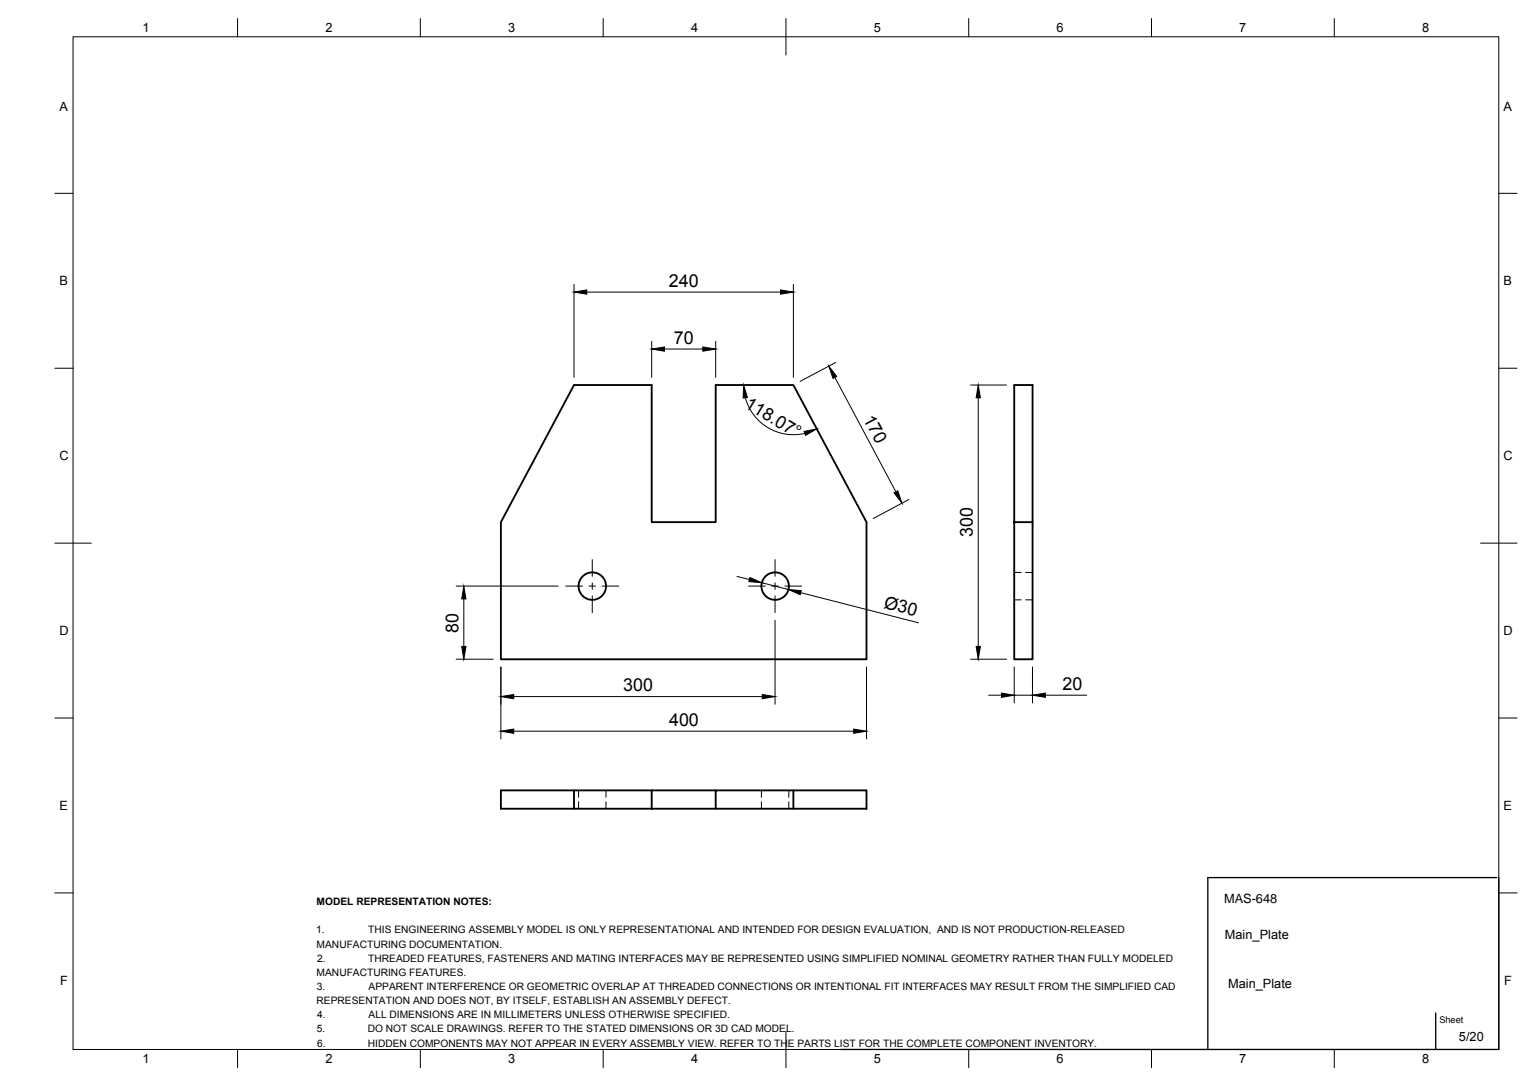
ISO-10303-21;
HEADER;
FILE_DESCRIPTION((''),'2;1');
FILE_NAME('Main_Plate.step','2026-10-09T12:47:58-07:00',(''),(''),'','','');
FILE_SCHEMA (('AUTOMOTIVE_DESIGN { 1 0 10303 214 3 1 1 }'));
ENDSEC;
DATA;
#10=MECHANICAL_DESIGN_GEOMETRIC_PRESENTATION_REPRESENTATION('',(#312),#3475);
#143=FACE_BOUND('',#473,.T.) ;
#144=FACE_BOUND('',#474,.T.) ;
#145=FACE_BOUND('',#476,.T.) ;
#146=FACE_BOUND('',#477,.T.) ;
#168=CIRCLE('',#1990,15.) ;
#169=CIRCLE('',#1991,15.) ;
#170=CIRCLE('',#1993,15.) ;
#171=CIRCLE('',#1994,15.) ;
#257=CYLINDRICAL_SURFACE('',#1989,15.) ;
#258=CYLINDRICAL_SURFACE('',#1992,15.) ;
#288=SHAPE_REPRESENTATION_RELATIONSHIP('SRR','None',#3542,#300) ;
#300=ADVANCED_BREP_SHAPE_REPRESENTATION('',(#324),#3462) ;
#312=STYLED_ITEM('',(#3628),#324) ;
#324=MANIFOLD_SOLID_BREP('Body1',#1826) ;
#347=FACE_OUTER_BOUND('',#463,.T.) ;
#348=FACE_OUTER_BOUND('',#464,.T.) ;
#349=FACE_OUTER_BOUND('',#465,.T.) ;
#350=FACE_OUTER_BOUND('',#466,.T.) ;
#351=FACE_OUTER_BOUND('',#467,.T.) ;
#352=FACE_OUTER_BOUND('',#468,.T.) ;
#353=FACE_OUTER_BOUND('',#469,.T.) ;
#354=FACE_OUTER_BOUND('',#470,.T.) ;
#355=FACE_OUTER_BOUND('',#471,.T.) ;
#356=FACE_OUTER_BOUND('',#472,.T.) ;
#357=FACE_OUTER_BOUND('',#475,.T.) ;
#358=FACE_OUTER_BOUND('',#478,.T.) ;
#359=FACE_OUTER_BOUND('',#479,.T.) ;
#360=FACE_OUTER_BOUND('',#480,.T.) ;
#463=EDGE_LOOP('',(#1248,#1249,#1250,#1251)) ;
#464=EDGE_LOOP('',(#1252,#1253,#1254,#1255)) ;
#465=EDGE_LOOP('',(#1256,#1257,#1258,#1259)) ;
#466=EDGE_LOOP('',(#1260,#1261,#1262,#1263)) ;
#467=EDGE_LOOP('',(#1264,#1265,#1266,#1267)) ;
#468=EDGE_LOOP('',(#1268,#1269,#1270,#1271)) ;
#469=EDGE_LOOP('',(#1272,#1273,#1274,#1275)) ;
#470=EDGE_LOOP('',(#1276,#1277,#1278,#1279)) ;
#471=EDGE_LOOP('',(#1280,#1281,#1282,#1283)) ;
#472=EDGE_LOOP('',(#1284,#1285,#1286,#1287,#1288,#1289,#1290,#1291,#1292,
#1293)) ;
#473=EDGE_LOOP('',(#1294)) ;
#474=EDGE_LOOP('',(#1295)) ;
#475=EDGE_LOOP('',(#1296,#1297,#1298,#1299,#1300,#1301,#1302,#1303,#1304,
#1305)) ;
#476=EDGE_LOOP('',(#1306)) ;
#477=EDGE_LOOP('',(#1307)) ;
#478=EDGE_LOOP('',(#1308,#1309,#1310,#1311)) ;
#479=EDGE_LOOP('',(#1312,#1313,#1314,#1315)) ;
#480=EDGE_LOOP('',(#1316,#1317,#1318,#1319)) ;
#612=LINE('',#2890,#731) ;
#613=LINE('',#2896,#732) ;
#614=LINE('',#2901,#733) ;
#615=LINE('',#2903,#734) ;
#616=LINE('',#2905,#735) ;
#617=LINE('',#2906,#736) ;
#618=LINE('',#2910,#737) ;
#619=LINE('',#2912,#738) ;
#620=LINE('',#2914,#739) ;
#621=LINE('',#2915,#740) ;
#622=LINE('',#2918,#741) ;
#623=LINE('',#2920,#742) ;
#624=LINE('',#2921,#743) ;
#625=LINE('',#2924,#744) ;
#626=LINE('',#2926,#745) ;
#627=LINE('',#2927,#746) ;
#628=LINE('',#2930,#747) ;
#629=LINE('',#2932,#748) ;
#630=LINE('',#2933,#749) ;
#631=LINE('',#2937,#750) ;
#632=LINE('',#2938,#751) ;
#633=LINE('',#2939,#752) ;
#634=LINE('',#2941,#753) ;
#635=LINE('',#2942,#754) ;
#636=LINE('',#2946,#755) ;
#637=LINE('',#2947,#756) ;
#638=LINE('',#2948,#757) ;
#639=LINE('',#2951,#758) ;
#640=LINE('',#2953,#759) ;
#641=LINE('',#2954,#760) ;
#642=LINE('',#2956,#761) ;
#643=LINE('',#2957,#762) ;
#731=VECTOR('',#2283,15.) ;
#732=VECTOR('',#2290,15.) ;
#733=VECTOR('',#2295,1000.) ;
#734=VECTOR('',#2296,1000.) ;
#735=VECTOR('',#2297,1000.) ;
#736=VECTOR('',#2298,1000.) ;
#737=VECTOR('',#2301,1000.) ;
#738=VECTOR('',#2302,1000.) ;
#739=VECTOR('',#2303,1000.) ;
#740=VECTOR('',#2304,1000.) ;
#741=VECTOR('',#2307,1000.) ;
#742=VECTOR('',#2308,1000.) ;
#743=VECTOR('',#2309,1000.) ;
#744=VECTOR('',#2312,1000.) ;
#745=VECTOR('',#2313,1000.) ;
#746=VECTOR('',#2314,1000.) ;
#747=VECTOR('',#2317,1000.) ;
#748=VECTOR('',#2318,1000.) ;
#749=VECTOR('',#2319,1000.) ;
#750=VECTOR('',#2322,1000.) ;
#751=VECTOR('',#2323,1000.) ;
#752=VECTOR('',#2324,1000.) ;
#753=VECTOR('',#2327,1000.) ;
#754=VECTOR('',#2328,1000.) ;
#755=VECTOR('',#2331,1000.) ;
#756=VECTOR('',#2332,1000.) ;
#757=VECTOR('',#2333,1000.) ;
#758=VECTOR('',#2336,1000.) ;
#759=VECTOR('',#2337,1000.) ;
#760=VECTOR('',#2338,1000.) ;
#761=VECTOR('',#2341,1000.) ;
#762=VECTOR('',#2342,1000.) ;
#843=VERTEX_POINT('',#2887) ;
#844=VERTEX_POINT('',#2889) ;
#845=VERTEX_POINT('',#2893) ;
#846=VERTEX_POINT('',#2895) ;
#847=VERTEX_POINT('',#2899) ;
#848=VERTEX_POINT('',#2900) ;
#849=VERTEX_POINT('',#2902) ;
#850=VERTEX_POINT('',#2904) ;
#851=VERTEX_POINT('',#2908) ;
#852=VERTEX_POINT('',#2909) ;
#853=VERTEX_POINT('',#2911) ;
#854=VERTEX_POINT('',#2913) ;
#855=VERTEX_POINT('',#2917) ;
#856=VERTEX_POINT('',#2919) ;
#857=VERTEX_POINT('',#2923) ;
#858=VERTEX_POINT('',#2925) ;
#859=VERTEX_POINT('',#2929) ;
#860=VERTEX_POINT('',#2931) ;
#861=VERTEX_POINT('',#2935) ;
#862=VERTEX_POINT('',#2936) ;
#863=VERTEX_POINT('',#2944) ;
#864=VERTEX_POINT('',#2945) ;
#865=VERTEX_POINT('',#2950) ;
#866=VERTEX_POINT('',#2952) ;
#996=EDGE_CURVE('',#843,#843,#168,.T.) ;
#997=EDGE_CURVE('',#843,#844,#612,.T.) ;
#998=EDGE_CURVE('',#844,#844,#169,.T.) ;
#999=EDGE_CURVE('',#845,#845,#170,.T.) ;
#1000=EDGE_CURVE('',#845,#846,#613,.T.) ;
#1001=EDGE_CURVE('',#846,#846,#171,.T.) ;
#1002=EDGE_CURVE('',#847,#848,#614,.T.) ;
#1003=EDGE_CURVE('',#849,#847,#615,.T.) ;
#1004=EDGE_CURVE('',#850,#849,#616,.T.) ;
#1005=EDGE_CURVE('',#850,#848,#617,.T.) ;
#1006=EDGE_CURVE('',#851,#852,#618,.T.) ;
#1007=EDGE_CURVE('',#853,#851,#619,.T.) ;
#1008=EDGE_CURVE('',#853,#854,#620,.T.) ;
#1009=EDGE_CURVE('',#854,#852,#621,.T.) ;
#1010=EDGE_CURVE('',#855,#851,#622,.T.) ;
#1011=EDGE_CURVE('',#856,#855,#623,.T.) ;
#1012=EDGE_CURVE('',#856,#853,#624,.T.) ;
#1013=EDGE_CURVE('',#857,#855,#625,.T.) ;
#1014=EDGE_CURVE('',#858,#857,#626,.T.) ;
#1015=EDGE_CURVE('',#858,#856,#627,.T.) ;
#1016=EDGE_CURVE('',#859,#857,#628,.T.) ;
#1017=EDGE_CURVE('',#860,#859,#629,.T.) ;
#1018=EDGE_CURVE('',#860,#858,#630,.T.) ;
#1019=EDGE_CURVE('',#861,#862,#631,.T.) ;
#1020=EDGE_CURVE('',#861,#860,#632,.T.) ;
#1021=EDGE_CURVE('',#862,#859,#633,.T.) ;
#1022=EDGE_CURVE('',#852,#849,#634,.T.) ;
#1023=EDGE_CURVE('',#854,#850,#635,.T.) ;
#1024=EDGE_CURVE('',#863,#864,#636,.T.) ;
#1025=EDGE_CURVE('',#864,#848,#637,.T.) ;
#1026=EDGE_CURVE('',#861,#863,#638,.T.) ;
#1027=EDGE_CURVE('',#865,#847,#639,.T.) ;
#1028=EDGE_CURVE('',#866,#865,#640,.T.) ;
#1029=EDGE_CURVE('',#862,#866,#641,.T.) ;
#1030=EDGE_CURVE('',#863,#866,#642,.T.) ;
#1031=EDGE_CURVE('',#864,#865,#643,.T.) ;
#1248=ORIENTED_EDGE('',*,*,#996,.F.) ;
#1249=ORIENTED_EDGE('',*,*,#997,.T.) ;
#1250=ORIENTED_EDGE('',*,*,#998,.T.) ;
#1251=ORIENTED_EDGE('',*,*,#997,.F.) ;
#1252=ORIENTED_EDGE('',*,*,#999,.F.) ;
#1253=ORIENTED_EDGE('',*,*,#1000,.T.) ;
#1254=ORIENTED_EDGE('',*,*,#1001,.T.) ;
#1255=ORIENTED_EDGE('',*,*,#1000,.F.) ;
#1256=ORIENTED_EDGE('',*,*,#1002,.F.) ;
#1257=ORIENTED_EDGE('',*,*,#1003,.F.) ;
#1258=ORIENTED_EDGE('',*,*,#1004,.F.) ;
#1259=ORIENTED_EDGE('',*,*,#1005,.T.) ;
#1260=ORIENTED_EDGE('',*,*,#1006,.F.) ;
#1261=ORIENTED_EDGE('',*,*,#1007,.F.) ;
#1262=ORIENTED_EDGE('',*,*,#1008,.T.) ;
#1263=ORIENTED_EDGE('',*,*,#1009,.T.) ;
#1264=ORIENTED_EDGE('',*,*,#1010,.F.) ;
#1265=ORIENTED_EDGE('',*,*,#1011,.F.) ;
#1266=ORIENTED_EDGE('',*,*,#1012,.T.) ;
#1267=ORIENTED_EDGE('',*,*,#1007,.T.) ;
#1268=ORIENTED_EDGE('',*,*,#1013,.F.) ;
#1269=ORIENTED_EDGE('',*,*,#1014,.F.) ;
#1270=ORIENTED_EDGE('',*,*,#1015,.T.) ;
#1271=ORIENTED_EDGE('',*,*,#1011,.T.) ;
#1272=ORIENTED_EDGE('',*,*,#1016,.F.) ;
#1273=ORIENTED_EDGE('',*,*,#1017,.F.) ;
#1274=ORIENTED_EDGE('',*,*,#1018,.T.) ;
#1275=ORIENTED_EDGE('',*,*,#1014,.T.) ;
#1276=ORIENTED_EDGE('',*,*,#1019,.F.) ;
#1277=ORIENTED_EDGE('',*,*,#1020,.T.) ;
#1278=ORIENTED_EDGE('',*,*,#1017,.T.) ;
#1279=ORIENTED_EDGE('',*,*,#1021,.F.) ;
#1280=ORIENTED_EDGE('',*,*,#1022,.F.) ;
#1281=ORIENTED_EDGE('',*,*,#1009,.F.) ;
#1282=ORIENTED_EDGE('',*,*,#1023,.T.) ;
#1283=ORIENTED_EDGE('',*,*,#1004,.T.) ;
#1284=ORIENTED_EDGE('',*,*,#1024,.T.) ;
#1285=ORIENTED_EDGE('',*,*,#1025,.T.) ;
#1286=ORIENTED_EDGE('',*,*,#1005,.F.) ;
#1287=ORIENTED_EDGE('',*,*,#1023,.F.) ;
#1288=ORIENTED_EDGE('',*,*,#1008,.F.) ;
#1289=ORIENTED_EDGE('',*,*,#1012,.F.) ;
#1290=ORIENTED_EDGE('',*,*,#1015,.F.) ;
#1291=ORIENTED_EDGE('',*,*,#1018,.F.) ;
#1292=ORIENTED_EDGE('',*,*,#1020,.F.) ;
#1293=ORIENTED_EDGE('',*,*,#1026,.T.) ;
#1294=ORIENTED_EDGE('',*,*,#996,.T.) ;
#1295=ORIENTED_EDGE('',*,*,#999,.T.) ;
#1296=ORIENTED_EDGE('',*,*,#1027,.F.) ;
#1297=ORIENTED_EDGE('',*,*,#1028,.F.) ;
#1298=ORIENTED_EDGE('',*,*,#1029,.F.) ;
#1299=ORIENTED_EDGE('',*,*,#1021,.T.) ;
#1300=ORIENTED_EDGE('',*,*,#1016,.T.) ;
#1301=ORIENTED_EDGE('',*,*,#1013,.T.) ;
#1302=ORIENTED_EDGE('',*,*,#1010,.T.) ;
#1303=ORIENTED_EDGE('',*,*,#1006,.T.) ;
#1304=ORIENTED_EDGE('',*,*,#1022,.T.) ;
#1305=ORIENTED_EDGE('',*,*,#1003,.T.) ;
#1306=ORIENTED_EDGE('',*,*,#998,.F.) ;
#1307=ORIENTED_EDGE('',*,*,#1001,.F.) ;
#1308=ORIENTED_EDGE('',*,*,#1030,.T.) ;
#1309=ORIENTED_EDGE('',*,*,#1028,.T.) ;
#1310=ORIENTED_EDGE('',*,*,#1031,.F.) ;
#1311=ORIENTED_EDGE('',*,*,#1024,.F.) ;
#1312=ORIENTED_EDGE('',*,*,#1002,.T.) ;
#1313=ORIENTED_EDGE('',*,*,#1025,.F.) ;
#1314=ORIENTED_EDGE('',*,*,#1031,.T.) ;
#1315=ORIENTED_EDGE('',*,*,#1027,.T.) ;
#1316=ORIENTED_EDGE('',*,*,#1019,.T.) ;
#1317=ORIENTED_EDGE('',*,*,#1029,.T.) ;
#1318=ORIENTED_EDGE('',*,*,#1030,.F.) ;
#1319=ORIENTED_EDGE('',*,*,#1026,.F.) ;
#1656=PLANE('',#1995) ;
#1657=PLANE('',#1996) ;
#1658=PLANE('',#1997) ;
#1659=PLANE('',#1998) ;
#1660=PLANE('',#1999) ;
#1661=PLANE('',#2000) ;
#1662=PLANE('',#2001) ;
#1663=PLANE('',#2002) ;
#1664=PLANE('',#2003) ;
#1665=PLANE('',#2004) ;
#1666=PLANE('',#2005) ;
#1667=PLANE('',#2006) ;
#1723=ADVANCED_FACE('',(#347),#257,.F.) ;
#1724=ADVANCED_FACE('',(#348),#258,.F.) ;
#1725=ADVANCED_FACE('',(#349),#1656,.T.) ;
#1726=ADVANCED_FACE('',(#350),#1657,.T.) ;
#1727=ADVANCED_FACE('',(#351),#1658,.T.) ;
#1728=ADVANCED_FACE('',(#352),#1659,.T.) ;
#1729=ADVANCED_FACE('',(#353),#1660,.T.) ;
#1730=ADVANCED_FACE('',(#354),#1661,.T.) ;
#1731=ADVANCED_FACE('',(#355),#1662,.T.) ;
#1732=ADVANCED_FACE('',(#356,#143,#144),#1663,.F.) ;
#1733=ADVANCED_FACE('',(#357,#145,#146),#1664,.T.) ;
#1734=ADVANCED_FACE('',(#358),#1665,.F.) ;
#1735=ADVANCED_FACE('',(#359),#1666,.F.) ;
#1736=ADVANCED_FACE('',(#360),#1667,.F.) ;
#1826=CLOSED_SHELL('',(#1723,#1724,#1725,#1726,#1727,#1728,#1729,#1730,
#1731,#1732,#1733,#1734,#1735,#1736)) ;
#1988=AXIS2_PLACEMENT_3D('',#2885,#2277,#2278) ;
#1989=AXIS2_PLACEMENT_3D('',#2886,#2279,#2280) ;
#1990=AXIS2_PLACEMENT_3D('',#2888,#2281,#2282) ;
#1991=AXIS2_PLACEMENT_3D('',#2891,#2284,#2285) ;
#1992=AXIS2_PLACEMENT_3D('',#2892,#2286,#2287) ;
#1993=AXIS2_PLACEMENT_3D('',#2894,#2288,#2289) ;
#1994=AXIS2_PLACEMENT_3D('',#2897,#2291,#2292) ;
#1995=AXIS2_PLACEMENT_3D('',#2898,#2293,#2294) ;
#1996=AXIS2_PLACEMENT_3D('',#2907,#2299,#2300) ;
#1997=AXIS2_PLACEMENT_3D('',#2916,#2305,#2306) ;
#1998=AXIS2_PLACEMENT_3D('',#2922,#2310,#2311) ;
#1999=AXIS2_PLACEMENT_3D('',#2928,#2315,#2316) ;
#2000=AXIS2_PLACEMENT_3D('',#2934,#2320,#2321) ;
#2001=AXIS2_PLACEMENT_3D('',#2940,#2325,#2326) ;
#2002=AXIS2_PLACEMENT_3D('',#2943,#2329,#2330) ;
#2003=AXIS2_PLACEMENT_3D('',#2949,#2334,#2335) ;
#2004=AXIS2_PLACEMENT_3D('',#2955,#2339,#2340) ;
#2005=AXIS2_PLACEMENT_3D('',#2958,#2343,#2344) ;
#2006=AXIS2_PLACEMENT_3D('',#2959,#2345,#2346) ;
#2277=DIRECTION('axis',(0.,0.,1.)) ;
#2278=DIRECTION('refdir',(1.,0.,0.)) ;
#2279=DIRECTION('center_axis',(0.,0.,1.)) ;
#2280=DIRECTION('ref_axis',(1.,0.,0.)) ;
#2281=DIRECTION('center_axis',(0.,0.,1.)) ;
#2282=DIRECTION('ref_axis',(1.,0.,0.)) ;
#2283=DIRECTION('',(0.,0.,1.)) ;
#2284=DIRECTION('center_axis',(0.,0.,1.)) ;
#2285=DIRECTION('ref_axis',(1.,0.,0.)) ;
#2286=DIRECTION('center_axis',(0.,0.,1.)) ;
#2287=DIRECTION('ref_axis',(1.,0.,0.)) ;
#2288=DIRECTION('center_axis',(0.,0.,1.)) ;
#2289=DIRECTION('ref_axis',(1.,0.,0.)) ;
#2290=DIRECTION('',(0.,0.,1.)) ;
#2291=DIRECTION('center_axis',(0.,0.,1.)) ;
#2292=DIRECTION('ref_axis',(-1.,0.,0.)) ;
#2293=DIRECTION('center_axis',(-2.31296463463574E-16,1.,0.)) ;
#2294=DIRECTION('ref_axis',(-1.,-2.31296463463574E-16,0.)) ;
#2295=DIRECTION('',(0.,0.,-1.)) ;
#2296=DIRECTION('',(-1.,-2.31296463463574E-16,0.)) ;
#2297=DIRECTION('',(0.,0.,1.)) ;
#2298=DIRECTION('',(-1.,-2.31296463463574E-16,0.)) ;
#2299=DIRECTION('center_axis',(1.,0.,0.)) ;
#2300=DIRECTION('ref_axis',(0.,0.,-1.)) ;
#2301=DIRECTION('',(0.,1.,0.)) ;
#2302=DIRECTION('',(0.,0.,1.)) ;
#2303=DIRECTION('',(0.,1.,0.)) ;
#2304=DIRECTION('',(0.,0.,1.)) ;
#2305=DIRECTION('center_axis',(0.,-1.,0.)) ;
#2306=DIRECTION('ref_axis',(0.,0.,-1.)) ;
#2307=DIRECTION('',(1.,0.,0.)) ;
#2308=DIRECTION('',(0.,0.,1.)) ;
#2309=DIRECTION('',(1.,0.,0.)) ;
#2310=DIRECTION('center_axis',(-1.,0.,0.)) ;
#2311=DIRECTION('ref_axis',(0.,0.,1.)) ;
#2312=DIRECTION('',(0.,-1.,0.)) ;
#2313=DIRECTION('',(0.,0.,1.)) ;
#2314=DIRECTION('',(0.,-1.,0.)) ;
#2315=DIRECTION('center_axis',(-0.882352941176471,0.470588235294118,0.)) ;
#2316=DIRECTION('ref_axis',(-0.470588235294118,-0.882352941176471,0.)) ;
#2317=DIRECTION('',(-0.470588235294118,-0.88235294117647,0.)) ;
#2318=DIRECTION('',(0.,0.,1.)) ;
#2319=DIRECTION('',(-0.470588235294118,-0.88235294117647,0.)) ;
#2320=DIRECTION('center_axis',(-2.31296463463574E-16,1.,0.)) ;
#2321=DIRECTION('ref_axis',(-1.,-2.31296463463574E-16,0.)) ;
#2322=DIRECTION('',(0.,0.,1.)) ;
#2323=DIRECTION('',(-1.,-2.31296463463574E-16,0.)) ;
#2324=DIRECTION('',(-1.,-2.31296463463574E-16,0.)) ;
#2325=DIRECTION('center_axis',(0.882352941176471,0.470588235294118,0.)) ;
#2326=DIRECTION('ref_axis',(-0.470588235294118,0.882352941176471,0.)) ;
#2327=DIRECTION('',(-0.470588235294118,0.882352941176471,0.)) ;
#2328=DIRECTION('',(-0.470588235294118,0.882352941176471,0.)) ;
#2329=DIRECTION('center_axis',(0.,0.,1.)) ;
#2330=DIRECTION('ref_axis',(1.,0.,0.)) ;
#2331=DIRECTION('',(1.,0.,0.)) ;
#2332=DIRECTION('',(0.,1.,0.)) ;
#2333=DIRECTION('',(9.25185853854297E-17,-1.,0.)) ;
#2334=DIRECTION('center_axis',(0.,0.,1.)) ;
#2335=DIRECTION('ref_axis',(1.,0.,0.)) ;
#2336=DIRECTION('',(0.,1.,0.)) ;
#2337=DIRECTION('',(1.,0.,0.)) ;
#2338=DIRECTION('',(9.25185853854297E-17,-1.,0.)) ;
#2339=DIRECTION('center_axis',(0.,-1.,0.)) ;
#2340=DIRECTION('ref_axis',(0.,0.,-1.)) ;
#2341=DIRECTION('',(0.,0.,1.)) ;
#2342=DIRECTION('',(0.,0.,1.)) ;
#2343=DIRECTION('center_axis',(1.,0.,0.)) ;
#2344=DIRECTION('ref_axis',(0.,0.,-1.)) ;
#2345=DIRECTION('center_axis',(-1.,-9.25185853854297E-17,0.)) ;
#2346=DIRECTION('ref_axis',(9.25185853854297E-17,-1.,0.)) ;
#2885=CARTESIAN_POINT('',(0.,0.,0.)) ;
#2886=CARTESIAN_POINT('Origin',(-300.,79.9999999999999,-22.)) ;
#2887=CARTESIAN_POINT('',(-315.,79.9999999999999,-20.)) ;
#2888=CARTESIAN_POINT('Origin',(-300.,79.9999999999999,-20.)) ;
#2889=CARTESIAN_POINT('',(-315.,79.9999999999999,0.)) ;
#2890=CARTESIAN_POINT('',(-315.,79.9999999999999,-22.)) ;
#2891=CARTESIAN_POINT('Origin',(-300.,79.9999999999999,0.)) ;
#2892=CARTESIAN_POINT('Origin',(-100.,79.9999999999999,-22.)) ;
#2893=CARTESIAN_POINT('',(-115.,79.9999999999999,-20.)) ;
#2894=CARTESIAN_POINT('Origin',(-100.,79.9999999999999,-20.)) ;
#2895=CARTESIAN_POINT('',(-115.,79.9999999999999,0.)) ;
#2896=CARTESIAN_POINT('',(-115.,79.9999999999999,-22.)) ;
#2897=CARTESIAN_POINT('Origin',(-100.,79.9999999999999,0.)) ;
#2898=CARTESIAN_POINT('Origin',(-80.,300.,-20.)) ;
#2899=CARTESIAN_POINT('',(-165.,300.,0.)) ;
#2900=CARTESIAN_POINT('',(-165.,300.,-20.)) ;
#2901=CARTESIAN_POINT('',(-165.,300.,-20.)) ;
#2902=CARTESIAN_POINT('',(-80.,300.,0.)) ;
#2903=CARTESIAN_POINT('',(-80.,300.,0.)) ;
#2904=CARTESIAN_POINT('',(-80.,300.,-20.)) ;
#2905=CARTESIAN_POINT('',(-80.,300.,-20.)) ;
#2906=CARTESIAN_POINT('',(-80.,300.,-20.)) ;
#2907=CARTESIAN_POINT('Origin',(0.,0.,-20.)) ;
#2908=CARTESIAN_POINT('',(0.,0.,0.)) ;
#2909=CARTESIAN_POINT('',(0.,150.,0.)) ;
#2910=CARTESIAN_POINT('',(0.,0.,0.)) ;
#2911=CARTESIAN_POINT('',(0.,0.,-20.)) ;
#2912=CARTESIAN_POINT('',(0.,0.,-20.)) ;
#2913=CARTESIAN_POINT('',(0.,150.,-20.)) ;
#2914=CARTESIAN_POINT('',(0.,0.,-20.)) ;
#2915=CARTESIAN_POINT('',(0.,150.,-20.)) ;
#2916=CARTESIAN_POINT('Origin',(0.,0.,-20.)) ;
#2917=CARTESIAN_POINT('',(-400.,0.,0.)) ;
#2918=CARTESIAN_POINT('',(0.,0.,0.)) ;
#2919=CARTESIAN_POINT('',(-400.,0.,-20.)) ;
#2920=CARTESIAN_POINT('',(-400.,0.,-20.)) ;
#2921=CARTESIAN_POINT('',(0.,0.,-20.)) ;
#2922=CARTESIAN_POINT('Origin',(-400.,0.,-20.)) ;
#2923=CARTESIAN_POINT('',(-400.,150.,0.)) ;
#2924=CARTESIAN_POINT('',(-400.,0.,0.)) ;
#2925=CARTESIAN_POINT('',(-400.,150.,-20.)) ;
#2926=CARTESIAN_POINT('',(-400.,150.,-20.)) ;
#2927=CARTESIAN_POINT('',(-400.,0.,-20.)) ;
#2928=CARTESIAN_POINT('Origin',(-400.,150.,-20.)) ;
#2929=CARTESIAN_POINT('',(-320.,300.,0.)) ;
#2930=CARTESIAN_POINT('',(-400.,150.,0.)) ;
#2931=CARTESIAN_POINT('',(-320.,300.,-20.)) ;
#2932=CARTESIAN_POINT('',(-320.,300.,-20.)) ;
#2933=CARTESIAN_POINT('',(-400.,150.,-20.)) ;
#2934=CARTESIAN_POINT('Origin',(-80.,300.,-20.)) ;
#2935=CARTESIAN_POINT('',(-235.,300.,-20.)) ;
#2936=CARTESIAN_POINT('',(-235.,300.,0.)) ;
#2937=CARTESIAN_POINT('',(-235.,300.,-20.)) ;
#2938=CARTESIAN_POINT('',(-80.,300.,-20.)) ;
#2939=CARTESIAN_POINT('',(-80.,300.,0.)) ;
#2940=CARTESIAN_POINT('Origin',(0.,150.,-20.)) ;
#2941=CARTESIAN_POINT('',(0.,150.,0.)) ;
#2942=CARTESIAN_POINT('',(0.,150.,-20.)) ;
#2943=CARTESIAN_POINT('Origin',(0.,0.,-20.)) ;
#2944=CARTESIAN_POINT('',(-235.,150.,-20.)) ;
#2945=CARTESIAN_POINT('',(-165.,150.,-20.)) ;
#2946=CARTESIAN_POINT('',(0.,150.,-20.)) ;
#2947=CARTESIAN_POINT('',(-165.,0.,-20.)) ;
#2948=CARTESIAN_POINT('',(-235.,-2.1741867565576E-14,-20.)) ;
#2949=CARTESIAN_POINT('Origin',(0.,0.,0.)) ;
#2950=CARTESIAN_POINT('',(-165.,150.,0.)) ;
#2951=CARTESIAN_POINT('',(-165.,450.,0.)) ;
#2952=CARTESIAN_POINT('',(-235.,150.,0.)) ;
#2953=CARTESIAN_POINT('',(-235.,150.,0.)) ;
#2954=CARTESIAN_POINT('',(-235.,-2.1741867565576E-14,0.)) ;
#2955=CARTESIAN_POINT('Origin',(-235.,150.,-22.)) ;
#2956=CARTESIAN_POINT('',(-235.,150.,-22.)) ;
#2957=CARTESIAN_POINT('',(-165.,150.,-22.)) ;
#2958=CARTESIAN_POINT('Origin',(-165.,450.,-22.)) ;
#2959=CARTESIAN_POINT('Origin',(-235.,450.,-22.)) ;
#3444=UNCERTAINTY_MEASURE_WITH_UNIT(LENGTH_MEASURE(0.01),#3476,
'DISTANCE_ACCURACY_VALUE',
'Maximum model space distance between geometric entities at asserted c
onnectivities') ;
#3457=UNCERTAINTY_MEASURE_WITH_UNIT(LENGTH_MEASURE(0.01),#3476,
'DISTANCE_ACCURACY_VALUE',
'Maximum model space distance between geometric entities at asserted c
onnectivities') ;
#3462=(
GEOMETRIC_REPRESENTATION_CONTEXT(3)
GLOBAL_UNCERTAINTY_ASSIGNED_CONTEXT((#3444))
GLOBAL_UNIT_ASSIGNED_CONTEXT((#3476,#3478,#3479))
REPRESENTATION_CONTEXT('','3D')
) ;
#3475=(
GEOMETRIC_REPRESENTATION_CONTEXT(3)
GLOBAL_UNCERTAINTY_ASSIGNED_CONTEXT((#3457))
GLOBAL_UNIT_ASSIGNED_CONTEXT((#3476,#3478,#3479))
REPRESENTATION_CONTEXT('','3D')
) ;
#3476=(
LENGTH_UNIT()
NAMED_UNIT(*)
SI_UNIT(.MILLI.,.METRE.)
) ;
#3478=(
NAMED_UNIT(*)
PLANE_ANGLE_UNIT()
SI_UNIT($,.RADIAN.)
) ;
#3479=(
NAMED_UNIT(*)
SI_UNIT($,.STERADIAN.)
SOLID_ANGLE_UNIT()
) ;
#3484=SHAPE_DEFINITION_REPRESENTATION(#3501,#3542) ;
#3501=PRODUCT_DEFINITION_SHAPE('',$,#3560) ;
#3542=SHAPE_REPRESENTATION('',(#1988),#3462) ;
#3555=PRODUCT_DEFINITION_CONTEXT('part definition',#3608,'design') ;
#3560=PRODUCT_DEFINITION('Main_Plate',
'Main_Plate',#3577,#3555) ;
#3577=PRODUCT_DEFINITION_FORMATION('',$,#3614) ;
#3608=APPLICATION_CONTEXT(
'Core Data for Automotive Mechanical Design Process') ;
#3609=PRODUCT_CONTEXT('part definition',#3608,'mechanical') ;
#3614=PRODUCT('Main_Plate','Main_Plate',
$,(#3609)) ;
#3628=PRESENTATION_STYLE_ASSIGNMENT((#3630)) ;
#3630=SURFACE_STYLE_USAGE(.BOTH.,#3632) ;
#3632=SURFACE_SIDE_STYLE('',(#3634)) ;
#3634=SURFACE_STYLE_FILL_AREA(#3636) ;
#3636=FILL_AREA_STYLE('Opaque(202,209,238)',(#3638)) ;
#3638=FILL_AREA_STYLE_COLOUR('Opaque(202,209,238)',#3640) ;
#3640=COLOUR_RGB('Opaque(202,209,238)', 0.09019608, 0.27058824, 0.51372549) ;
ENDSEC;
END-ISO-10303-21;
